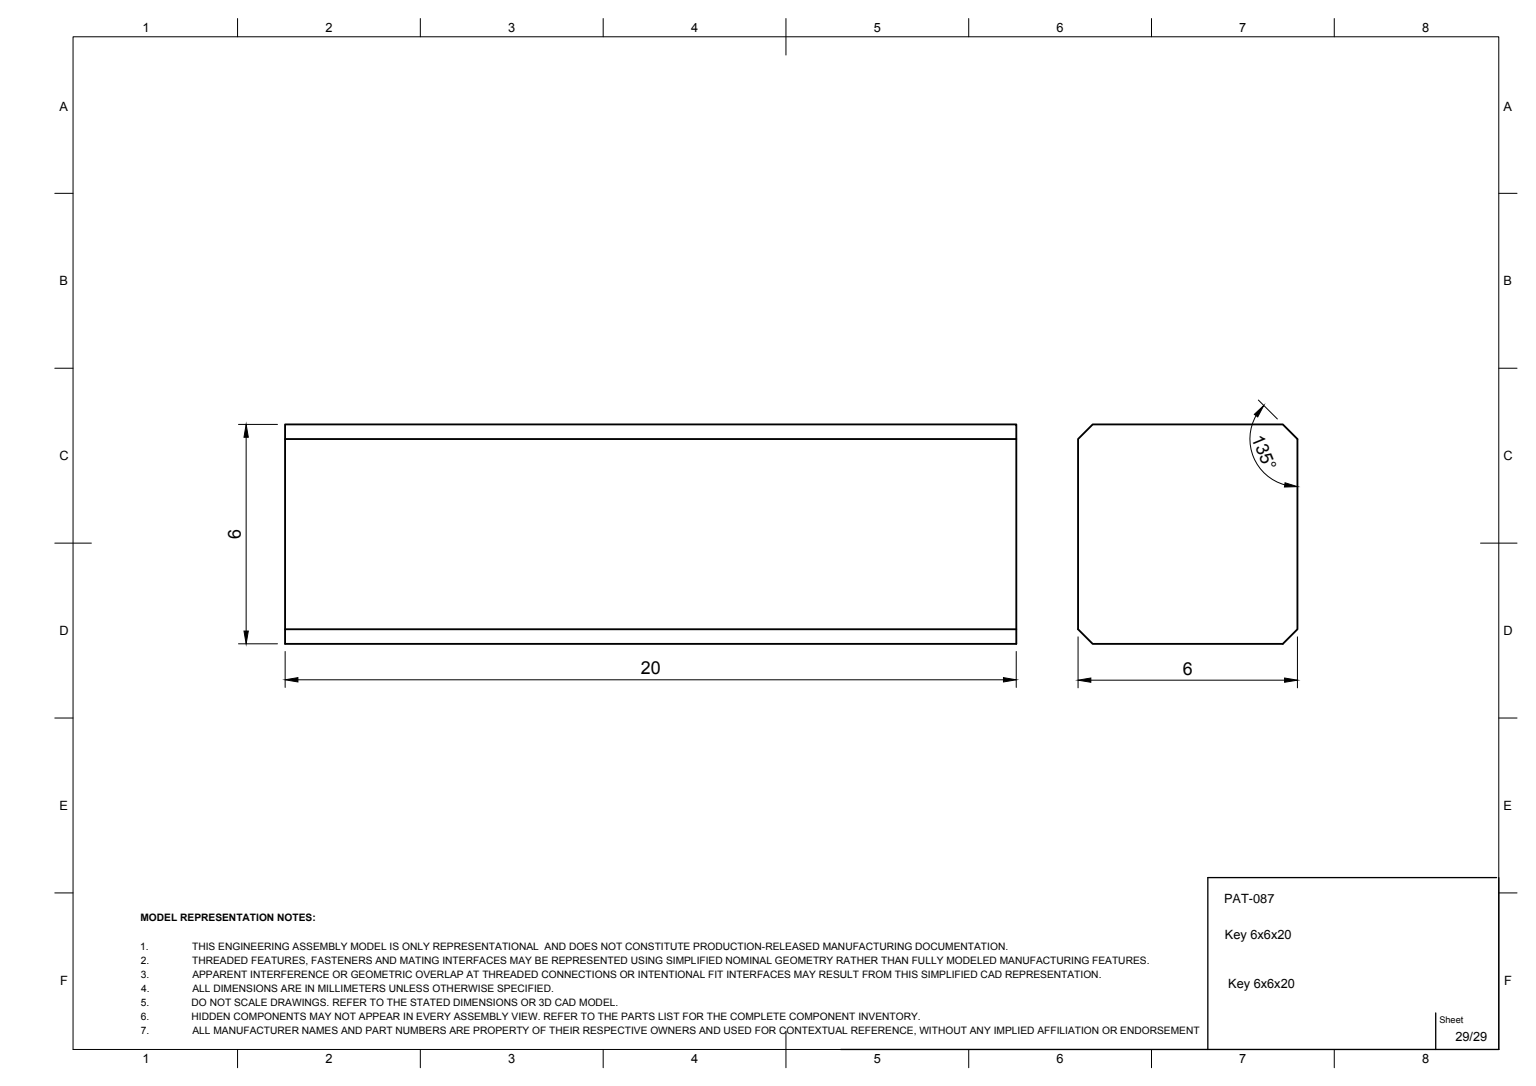
ISO-10303-21;
HEADER;
/* Generated by software containing ST-Developer
 * from STEP Tools, Inc. (www.steptools.com) 
 */

FILE_DESCRIPTION(
/* description */ ('Rigid flange shaft coupling assembly'),
/* implementation_level */ '2;1');

FILE_NAME(
/* name */ 'Key 6x6x20.step',
/* time_stamp */ '2026-10-27T10:47:16-07:00',
/* author */ (''),
/* organization */ (''),
/* preprocessor_version */ 'ST-DEVELOPER v20.2',
/* originating_system */ 'Autodesk Translation Framework v15.17.0.0',
/* authorisation */ '');

FILE_SCHEMA (('AUTOMOTIVE_DESIGN { 1 0 10303 214 3 1 1 }'));
ENDSEC;

DATA;
#10=MECHANICAL_DESIGN_GEOMETRIC_PRESENTATION_REPRESENTATION('',(#421),#9141);
#364=SHAPE_REPRESENTATION_RELATIONSHIP('SRR','None',#9300,#392);
#392=ADVANCED_BREP_SHAPE_REPRESENTATION('',(#449),#9135);
#421=STYLED_ITEM('',(#9500),#449);
#449=MANIFOLD_SOLID_BREP('Body1',#4776);
#693=PLANE('',#5476);
#694=PLANE('',#5477);
#695=PLANE('',#5478);
#696=PLANE('',#5479);
#697=PLANE('',#5480);
#698=PLANE('',#5481);
#699=PLANE('',#5482);
#700=PLANE('',#5483);
#701=PLANE('',#5484);
#702=PLANE('',#5485);
#945=FACE_OUTER_BOUND('',#1327,.T.);
#946=FACE_OUTER_BOUND('',#1328,.T.);
#947=FACE_OUTER_BOUND('',#1329,.T.);
#948=FACE_OUTER_BOUND('',#1330,.T.);
#949=FACE_OUTER_BOUND('',#1331,.T.);
#950=FACE_OUTER_BOUND('',#1332,.T.);
#951=FACE_OUTER_BOUND('',#1333,.T.);
#952=FACE_OUTER_BOUND('',#1334,.T.);
#953=FACE_OUTER_BOUND('',#1335,.T.);
#954=FACE_OUTER_BOUND('',#1336,.T.);
#1327=EDGE_LOOP('',(#4111,#4112,#4113,#4114,#4115,#4116,#4117,#4118));
#1328=EDGE_LOOP('',(#4119,#4120,#4121,#4122));
#1329=EDGE_LOOP('',(#4123,#4124,#4125,#4126));
#1330=EDGE_LOOP('',(#4127,#4128,#4129,#4130));
#1331=EDGE_LOOP('',(#4131,#4132,#4133,#4134));
#1332=EDGE_LOOP('',(#4135,#4136,#4137,#4138,#4139,#4140,#4141,#4142));
#1333=EDGE_LOOP('',(#4143,#4144,#4145,#4146));
#1334=EDGE_LOOP('',(#4147,#4148,#4149,#4150));
#1335=EDGE_LOOP('',(#4151,#4152,#4153,#4154));
#1336=EDGE_LOOP('',(#4155,#4156,#4157,#4158));
#1646=LINE('',#8681,#1991);
#1647=LINE('',#8683,#1992);
#1648=LINE('',#8685,#1993);
#1649=LINE('',#8687,#1994);
#1650=LINE('',#8689,#1995);
#1651=LINE('',#8691,#1996);
#1652=LINE('',#8693,#1997);
#1653=LINE('',#8694,#1998);
#1654=LINE('',#8697,#1999);
#1655=LINE('',#8699,#2000);
#1656=LINE('',#8700,#2001);
#1657=LINE('',#8703,#2002);
#1658=LINE('',#8704,#2003);
#1659=LINE('',#8707,#2004);
#1660=LINE('',#8708,#2005);
#1661=LINE('',#8711,#2006);
#1662=LINE('',#8712,#2007);
#1663=LINE('',#8716,#2008);
#1664=LINE('',#8717,#2009);
#1665=LINE('',#8719,#2010);
#1666=LINE('',#8720,#2011);
#1667=LINE('',#8722,#2012);
#1668=LINE('',#8724,#2013);
#1669=LINE('',#8726,#2014);
#1991=VECTOR('',#6651,1.);
#1992=VECTOR('',#6652,1.);
#1993=VECTOR('',#6653,1.);
#1994=VECTOR('',#6654,1.);
#1995=VECTOR('',#6655,1.);
#1996=VECTOR('',#6656,1.);
#1997=VECTOR('',#6657,1.);
#1998=VECTOR('',#6658,1.);
#1999=VECTOR('',#6661,1.);
#2000=VECTOR('',#6662,1.);
#2001=VECTOR('',#6663,1.);
#2002=VECTOR('',#6666,1.);
#2003=VECTOR('',#6667,1.);
#2004=VECTOR('',#6670,1.);
#2005=VECTOR('',#6671,1.);
#2006=VECTOR('',#6674,1.);
#2007=VECTOR('',#6675,1.);
#2008=VECTOR('',#6678,1.);
#2009=VECTOR('',#6679,1.);
#2010=VECTOR('',#6680,1.);
#2011=VECTOR('',#6681,1.);
#2012=VECTOR('',#6684,1.);
#2013=VECTOR('',#6687,1.);
#2014=VECTOR('',#6690,1.);
#2573=VERTEX_POINT('',#8679);
#2574=VERTEX_POINT('',#8680);
#2575=VERTEX_POINT('',#8682);
#2576=VERTEX_POINT('',#8684);
#2577=VERTEX_POINT('',#8686);
#2578=VERTEX_POINT('',#8688);
#2579=VERTEX_POINT('',#8690);
#2580=VERTEX_POINT('',#8692);
#2581=VERTEX_POINT('',#8696);
#2582=VERTEX_POINT('',#8698);
#2583=VERTEX_POINT('',#8702);
#2584=VERTEX_POINT('',#8706);
#2585=VERTEX_POINT('',#8710);
#2586=VERTEX_POINT('',#8714);
#2587=VERTEX_POINT('',#8715);
#2588=VERTEX_POINT('',#8718);
#3099=EDGE_CURVE('',#2573,#2574,#1646,.T.);
#3100=EDGE_CURVE('',#2575,#2573,#1647,.T.);
#3101=EDGE_CURVE('',#2576,#2575,#1648,.T.);
#3102=EDGE_CURVE('',#2577,#2576,#1649,.T.);
#3103=EDGE_CURVE('',#2578,#2577,#1650,.T.);
#3104=EDGE_CURVE('',#2579,#2578,#1651,.T.);
#3105=EDGE_CURVE('',#2580,#2579,#1652,.T.);
#3106=EDGE_CURVE('',#2574,#2580,#1653,.T.);
#3107=EDGE_CURVE('',#2577,#2581,#1654,.T.);
#3108=EDGE_CURVE('',#2581,#2582,#1655,.T.);
#3109=EDGE_CURVE('',#2582,#2578,#1656,.T.);
#3110=EDGE_CURVE('',#2583,#2576,#1657,.T.);
#3111=EDGE_CURVE('',#2583,#2581,#1658,.T.);
#3112=EDGE_CURVE('',#2575,#2584,#1659,.T.);
#3113=EDGE_CURVE('',#2584,#2583,#1660,.T.);
#3114=EDGE_CURVE('',#2585,#2573,#1661,.T.);
#3115=EDGE_CURVE('',#2585,#2584,#1662,.T.);
#3116=EDGE_CURVE('',#2586,#2587,#1663,.T.);
#3117=EDGE_CURVE('',#2582,#2586,#1664,.T.);
#3118=EDGE_CURVE('',#2588,#2585,#1665,.T.);
#3119=EDGE_CURVE('',#2587,#2588,#1666,.T.);
#3120=EDGE_CURVE('',#2579,#2586,#1667,.T.);
#3121=EDGE_CURVE('',#2574,#2588,#1668,.T.);
#3122=EDGE_CURVE('',#2587,#2580,#1669,.T.);
#4111=ORIENTED_EDGE('',*,*,#3099,.F.);
#4112=ORIENTED_EDGE('',*,*,#3100,.F.);
#4113=ORIENTED_EDGE('',*,*,#3101,.F.);
#4114=ORIENTED_EDGE('',*,*,#3102,.F.);
#4115=ORIENTED_EDGE('',*,*,#3103,.F.);
#4116=ORIENTED_EDGE('',*,*,#3104,.F.);
#4117=ORIENTED_EDGE('',*,*,#3105,.F.);
#4118=ORIENTED_EDGE('',*,*,#3106,.F.);
#4119=ORIENTED_EDGE('',*,*,#3103,.T.);
#4120=ORIENTED_EDGE('',*,*,#3107,.T.);
#4121=ORIENTED_EDGE('',*,*,#3108,.T.);
#4122=ORIENTED_EDGE('',*,*,#3109,.T.);
#4123=ORIENTED_EDGE('',*,*,#3102,.T.);
#4124=ORIENTED_EDGE('',*,*,#3110,.F.);
#4125=ORIENTED_EDGE('',*,*,#3111,.T.);
#4126=ORIENTED_EDGE('',*,*,#3107,.F.);
#4127=ORIENTED_EDGE('',*,*,#3101,.T.);
#4128=ORIENTED_EDGE('',*,*,#3112,.T.);
#4129=ORIENTED_EDGE('',*,*,#3113,.T.);
#4130=ORIENTED_EDGE('',*,*,#3110,.T.);
#4131=ORIENTED_EDGE('',*,*,#3100,.T.);
#4132=ORIENTED_EDGE('',*,*,#3114,.F.);
#4133=ORIENTED_EDGE('',*,*,#3115,.T.);
#4134=ORIENTED_EDGE('',*,*,#3112,.F.);
#4135=ORIENTED_EDGE('',*,*,#3116,.F.);
#4136=ORIENTED_EDGE('',*,*,#3117,.F.);
#4137=ORIENTED_EDGE('',*,*,#3108,.F.);
#4138=ORIENTED_EDGE('',*,*,#3111,.F.);
#4139=ORIENTED_EDGE('',*,*,#3113,.F.);
#4140=ORIENTED_EDGE('',*,*,#3115,.F.);
#4141=ORIENTED_EDGE('',*,*,#3118,.F.);
#4142=ORIENTED_EDGE('',*,*,#3119,.F.);
#4143=ORIENTED_EDGE('',*,*,#3104,.T.);
#4144=ORIENTED_EDGE('',*,*,#3109,.F.);
#4145=ORIENTED_EDGE('',*,*,#3117,.T.);
#4146=ORIENTED_EDGE('',*,*,#3120,.F.);
#4147=ORIENTED_EDGE('',*,*,#3099,.T.);
#4148=ORIENTED_EDGE('',*,*,#3121,.T.);
#4149=ORIENTED_EDGE('',*,*,#3118,.T.);
#4150=ORIENTED_EDGE('',*,*,#3114,.T.);
#4151=ORIENTED_EDGE('',*,*,#3105,.T.);
#4152=ORIENTED_EDGE('',*,*,#3120,.T.);
#4153=ORIENTED_EDGE('',*,*,#3116,.T.);
#4154=ORIENTED_EDGE('',*,*,#3122,.T.);
#4155=ORIENTED_EDGE('',*,*,#3106,.T.);
#4156=ORIENTED_EDGE('',*,*,#3122,.F.);
#4157=ORIENTED_EDGE('',*,*,#3119,.T.);
#4158=ORIENTED_EDGE('',*,*,#3121,.F.);
#4681=ADVANCED_FACE('',(#945),#693,.F.);
#4682=ADVANCED_FACE('',(#946),#694,.T.);
#4683=ADVANCED_FACE('',(#947),#695,.T.);
#4684=ADVANCED_FACE('',(#948),#696,.T.);
#4685=ADVANCED_FACE('',(#949),#697,.T.);
#4686=ADVANCED_FACE('',(#950),#698,.T.);
#4687=ADVANCED_FACE('',(#951),#699,.F.);
#4688=ADVANCED_FACE('',(#952),#700,.T.);
#4689=ADVANCED_FACE('',(#953),#701,.T.);
#4690=ADVANCED_FACE('',(#954),#702,.T.);
#4776=CLOSED_SHELL('',(#4681,#4682,#4683,#4684,#4685,#4686,#4687,#4688,
#4689,#4690));
#5475=AXIS2_PLACEMENT_3D('',#8677,#6647,#6648);
#5476=AXIS2_PLACEMENT_3D('',#8678,#6649,#6650);
#5477=AXIS2_PLACEMENT_3D('',#8695,#6659,#6660);
#5478=AXIS2_PLACEMENT_3D('',#8701,#6664,#6665);
#5479=AXIS2_PLACEMENT_3D('',#8705,#6668,#6669);
#5480=AXIS2_PLACEMENT_3D('',#8709,#6672,#6673);
#5481=AXIS2_PLACEMENT_3D('',#8713,#6676,#6677);
#5482=AXIS2_PLACEMENT_3D('',#8721,#6682,#6683);
#5483=AXIS2_PLACEMENT_3D('',#8723,#6685,#6686);
#5484=AXIS2_PLACEMENT_3D('',#8725,#6688,#6689);
#5485=AXIS2_PLACEMENT_3D('',#8727,#6691,#6692);
#6647=DIRECTION('axis',(0.,0.,1.));
#6648=DIRECTION('refdir',(1.,0.,0.));
#6649=DIRECTION('center_axis',(1.,0.,0.));
#6650=DIRECTION('ref_axis',(0.,0.,-1.));
#6651=DIRECTION('',(0.,-0.707106781186547,-0.707106781186548));
#6652=DIRECTION('',(0.,-1.,0.));
#6653=DIRECTION('',(0.,-0.707106781186547,0.707106781186548));
#6654=DIRECTION('',(0.,0.,1.));
#6655=DIRECTION('',(0.,0.707106781186547,0.707106781186548));
#6656=DIRECTION('',(0.,1.,0.));
#6657=DIRECTION('',(0.,0.707106781186547,-0.707106781186548));
#6658=DIRECTION('',(0.,0.,-1.));
#6659=DIRECTION('center_axis',(0.,0.707106781186548,-0.707106781186547));
#6660=DIRECTION('ref_axis',(-1.,0.,0.));
#6661=DIRECTION('',(1.,0.,0.));
#6662=DIRECTION('',(0.,-0.707106781186547,-0.707106781186548));
#6663=DIRECTION('',(-1.,0.,0.));
#6664=DIRECTION('center_axis',(0.,1.,0.));
#6665=DIRECTION('ref_axis',(-1.,0.,0.));
#6666=DIRECTION('',(-1.,0.,0.));
#6667=DIRECTION('',(0.,0.,-1.));
#6668=DIRECTION('center_axis',(0.,0.707106781186548,0.707106781186547));
#6669=DIRECTION('ref_axis',(1.,0.,0.));
#6670=DIRECTION('',(1.,0.,0.));
#6671=DIRECTION('',(0.,0.707106781186547,-0.707106781186548));
#6672=DIRECTION('center_axis',(0.,0.,1.));
#6673=DIRECTION('ref_axis',(1.,0.,0.));
#6674=DIRECTION('',(-1.,0.,0.));
#6675=DIRECTION('',(0.,1.,0.));
#6676=DIRECTION('center_axis',(1.,0.,0.));
#6677=DIRECTION('ref_axis',(0.,0.,-1.));
#6678=DIRECTION('',(0.,-0.707106781186547,0.707106781186548));
#6679=DIRECTION('',(0.,-1.,0.));
#6680=DIRECTION('',(0.,0.707106781186547,0.707106781186548));
#6681=DIRECTION('',(0.,0.,1.));
#6682=DIRECTION('center_axis',(0.,0.,1.));
#6683=DIRECTION('ref_axis',(1.,0.,0.));
#6684=DIRECTION('',(1.,0.,0.));
#6685=DIRECTION('center_axis',(0.,-0.707106781186548,0.707106781186547));
#6686=DIRECTION('ref_axis',(1.,0.,0.));
#6687=DIRECTION('',(1.,0.,0.));
#6688=DIRECTION('center_axis',(0.,-0.707106781186548,-0.707106781186547));
#6689=DIRECTION('ref_axis',(-1.,0.,0.));
#6690=DIRECTION('',(-1.,0.,0.));
#6691=DIRECTION('center_axis',(0.,-1.,0.));
#6692=DIRECTION('ref_axis',(1.,0.,0.));
#8677=CARTESIAN_POINT('',(0.,0.,0.));
#8678=CARTESIAN_POINT('Origin',(-1.,0.,0.35));
#8679=CARTESIAN_POINT('',(-1.,-0.26,0.6));
#8680=CARTESIAN_POINT('',(-1.,-0.3,0.56));
#8681=CARTESIAN_POINT('',(-1.,-0.2675,0.5925));
#8682=CARTESIAN_POINT('',(-1.,0.26,0.6));
#8683=CARTESIAN_POINT('',(-1.,0.,0.6));
#8684=CARTESIAN_POINT('',(-1.,0.3,0.56));
#8685=CARTESIAN_POINT('',(-1.,0.2675,0.5925));
#8686=CARTESIAN_POINT('',(-1.,0.3,0.04));
#8687=CARTESIAN_POINT('',(-1.,0.3,0.175));
#8688=CARTESIAN_POINT('',(-1.,0.26,0.));
#8689=CARTESIAN_POINT('',(-1.,0.2925,0.0325));
#8690=CARTESIAN_POINT('',(-1.,-0.26,0.));
#8691=CARTESIAN_POINT('',(-1.,0.,0.));
#8692=CARTESIAN_POINT('',(-1.,-0.3,0.04));
#8693=CARTESIAN_POINT('',(-1.,-0.2925,0.0325));
#8694=CARTESIAN_POINT('',(-1.,-0.3,0.175));
#8695=CARTESIAN_POINT('Origin',(0.75,0.28,0.02));
#8696=CARTESIAN_POINT('',(1.,0.3,0.04));
#8697=CARTESIAN_POINT('',(0.75,0.3,0.04));
#8698=CARTESIAN_POINT('',(1.,0.26,0.));
#8699=CARTESIAN_POINT('',(1.,0.2925,0.0325));
#8700=CARTESIAN_POINT('',(0.75,0.26,0.));
#8701=CARTESIAN_POINT('Origin',(1.5,0.3,0.));
#8702=CARTESIAN_POINT('',(1.,0.3,0.56));
#8703=CARTESIAN_POINT('',(0.75,0.3,0.56));
#8704=CARTESIAN_POINT('',(1.,0.3,0.175));
#8705=CARTESIAN_POINT('Origin',(0.75,0.28,0.58));
#8706=CARTESIAN_POINT('',(1.,0.26,0.6));
#8707=CARTESIAN_POINT('',(0.75,0.26,0.6));
#8708=CARTESIAN_POINT('',(1.,0.2675,0.5925));
#8709=CARTESIAN_POINT('Origin',(0.,0.,0.6));
#8710=CARTESIAN_POINT('',(1.,-0.26,0.6));
#8711=CARTESIAN_POINT('',(-0.75,-0.26,0.6));
#8712=CARTESIAN_POINT('',(1.,0.,0.6));
#8713=CARTESIAN_POINT('Origin',(1.,0.,0.35));
#8714=CARTESIAN_POINT('',(1.,-0.26,0.));
#8715=CARTESIAN_POINT('',(1.,-0.3,0.04));
#8716=CARTESIAN_POINT('',(1.,-0.2925,0.0325));
#8717=CARTESIAN_POINT('',(1.,0.,0.));
#8718=CARTESIAN_POINT('',(1.,-0.3,0.56));
#8719=CARTESIAN_POINT('',(1.,-0.2675,0.5925));
#8720=CARTESIAN_POINT('',(1.,-0.3,0.175));
#8721=CARTESIAN_POINT('Origin',(0.,0.,0.));
#8722=CARTESIAN_POINT('',(-0.75,-0.26,0.));
#8723=CARTESIAN_POINT('Origin',(-0.75,-0.28,0.58));
#8724=CARTESIAN_POINT('',(-0.75,-0.3,0.56));
#8725=CARTESIAN_POINT('Origin',(-0.75,-0.28,0.02));
#8726=CARTESIAN_POINT('',(-0.75,-0.3,0.04));
#8727=CARTESIAN_POINT('Origin',(-1.5,-0.3,0.));
#9102=UNCERTAINTY_MEASURE_WITH_UNIT(LENGTH_MEASURE(0.001),#9142,
'DISTANCE_ACCURACY_VALUE',
'Maximum model space distance between geometric entities at asserted c
onnectivities');
#9108=UNCERTAINTY_MEASURE_WITH_UNIT(LENGTH_MEASURE(0.001),#9142,
'DISTANCE_ACCURACY_VALUE',
'Maximum model space distance between geometric entities at asserted c
onnectivities');
#9135=(
GEOMETRIC_REPRESENTATION_CONTEXT(3)
GLOBAL_UNCERTAINTY_ASSIGNED_CONTEXT((#9102))
GLOBAL_UNIT_ASSIGNED_CONTEXT((#9142,#9144,#9145))
REPRESENTATION_CONTEXT('','3D')
);
#9141=(
GEOMETRIC_REPRESENTATION_CONTEXT(3)
GLOBAL_UNCERTAINTY_ASSIGNED_CONTEXT((#9108))
GLOBAL_UNIT_ASSIGNED_CONTEXT((#9142,#9144,#9145))
REPRESENTATION_CONTEXT('','3D')
);
#9142=(
LENGTH_UNIT()
NAMED_UNIT(*)
SI_UNIT(.CENTI.,.METRE.)
);
#9144=(
NAMED_UNIT(*)
PLANE_ANGLE_UNIT()
SI_UNIT($,.RADIAN.)
);
#9145=(
NAMED_UNIT(*)
SI_UNIT($,.STERADIAN.)
SOLID_ANGLE_UNIT()
);
#9172=SHAPE_DEFINITION_REPRESENTATION(#9206,#9300);
#9206=PRODUCT_DEFINITION_SHAPE('',$,#9333);
#9300=SHAPE_REPRESENTATION('',(#5475),#9135);
#9306=PRODUCT_DEFINITION_CONTEXT('part definition',#9404,'design');
#9333=PRODUCT_DEFINITION('Key 6x6x20','Key 6x6x20',#9365,#9306);
#9365=PRODUCT_DEFINITION_FORMATION('',$,#9432);
#9404=APPLICATION_CONTEXT(
'Core Data for Automotive Mechanical Design Process');
#9405=PRODUCT_CONTEXT('part definition',#9404,'mechanical');
#9432=PRODUCT('Key 6x6x20','Key 6x6x20','Key 6x6x20',(#9405));
#9494=COLOUR_RGB('Grey',0.48,0.52,0.57);
#9495=FILL_AREA_STYLE_COLOUR('',#9494);
#9496=FILL_AREA_STYLE('',(#9495));
#9497=SURFACE_STYLE_FILL_AREA(#9496);
#9498=SURFACE_SIDE_STYLE('',(#9497));
#9499=SURFACE_STYLE_USAGE(.BOTH.,#9498);
#9500=PRESENTATION_STYLE_ASSIGNMENT((#9499));
ENDSEC;
END-ISO-10303-21;
